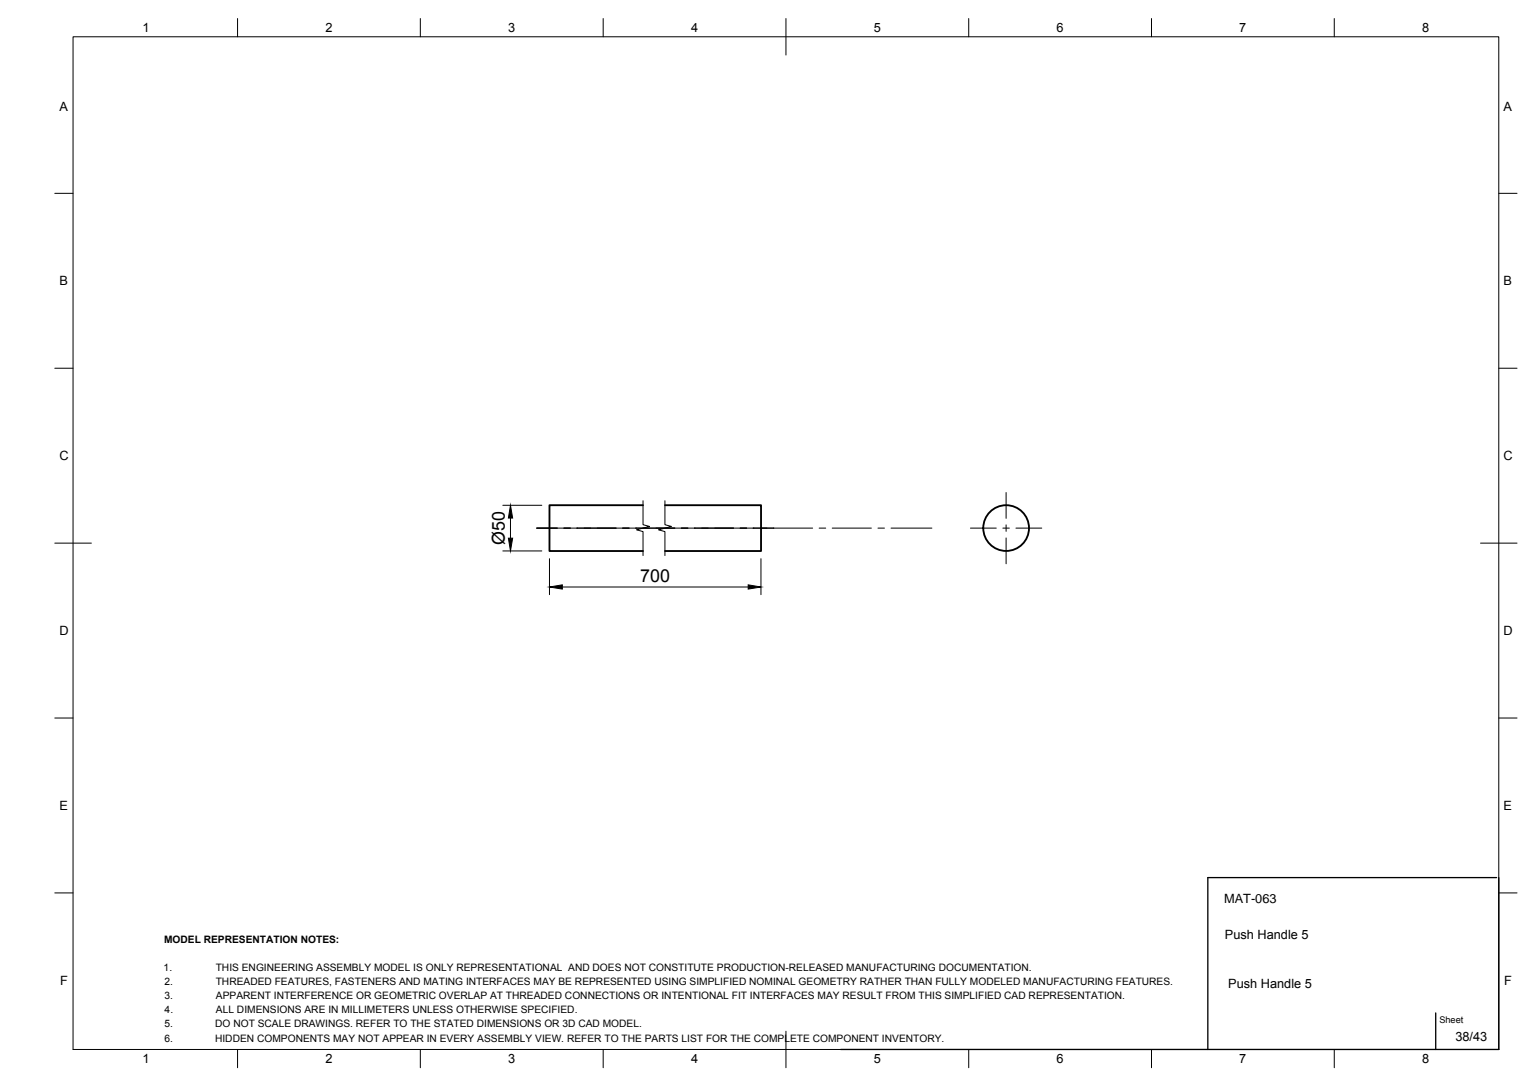
ISO-10303-21;
HEADER;
/* Generated by software containing ST-Developer
 * from STEP Tools, Inc. (www.steptools.com) 
 */

FILE_DESCRIPTION(
/* description */ (''),
/* implementation_level */ '2;1');

FILE_NAME(
/* name */ 'Push Handle 5.step',
/* time_stamp */ '2026-10-24T09:43:01-07:00',
/* author */ (''),
/* organization */ (''),
/* preprocessor_version */ 'ST-DEVELOPER v20.2',
/* originating_system */ 'Autodesk Translation Framework v15.15.0.0',
/* authorisation */ '');

FILE_SCHEMA (('AUTOMOTIVE_DESIGN { 1 0 10303 214 3 1 1 }'));
ENDSEC;

DATA;
#10=MECHANICAL_DESIGN_GEOMETRIC_PRESENTATION_REPRESENTATION('',(#301),#11112);
#235=SHAPE_REPRESENTATION_RELATIONSHIP('SRR','None',#11261,#268);
#268=ADVANCED_BREP_SHAPE_REPRESENTATION('',(#334),#11106);
#301=STYLED_ITEM('',(#11426),#334);
#334=MANIFOLD_SOLID_BREP('Push Handle 5',#6038);
#652=PLANE('',#7179);
#653=PLANE('',#7180);
#1010=FACE_OUTER_BOUND('',#1516,.T.);
#1011=FACE_OUTER_BOUND('',#1517,.T.);
#1012=FACE_OUTER_BOUND('',#1518,.T.);
#1516=EDGE_LOOP('',(#5403,#5404,#5405,#5406));
#1517=EDGE_LOOP('',(#5407));
#1518=EDGE_LOOP('',(#5408));
#1897=LINE('',#10903,#2256);
#2256=VECTOR('',#9141,0.025);
#2654=CIRCLE('',#7177,0.025);
#2655=CIRCLE('',#7178,0.025);
#3148=VERTEX_POINT('',#10900);
#3149=VERTEX_POINT('',#10902);
#3905=EDGE_CURVE('',#3148,#3148,#2654,.F.);
#3906=EDGE_CURVE('',#3148,#3149,#1897,.T.);
#3907=EDGE_CURVE('',#3149,#3149,#2655,.T.);
#5403=ORIENTED_EDGE('',*,*,#3905,.T.);
#5404=ORIENTED_EDGE('',*,*,#3906,.T.);
#5405=ORIENTED_EDGE('',*,*,#3907,.T.);
#5406=ORIENTED_EDGE('',*,*,#3906,.F.);
#5407=ORIENTED_EDGE('',*,*,#3907,.F.);
#5408=ORIENTED_EDGE('',*,*,#3905,.F.);
#5632=CYLINDRICAL_SURFACE('',#7176,0.025);
#5983=ADVANCED_FACE('',(#1010),#5632,.T.);
#5984=ADVANCED_FACE('',(#1011),#652,.T.);
#5985=ADVANCED_FACE('',(#1012),#653,.F.);
#6038=CLOSED_SHELL('',(#5983,#5984,#5985));
#7175=AXIS2_PLACEMENT_3D('',#10898,#9135,#9136);
#7176=AXIS2_PLACEMENT_3D('',#10899,#9137,#9138);
#7177=AXIS2_PLACEMENT_3D('',#10901,#9139,#9140);
#7178=AXIS2_PLACEMENT_3D('',#10904,#9142,#9143);
#7179=AXIS2_PLACEMENT_3D('',#10905,#9144,#9145);
#7180=AXIS2_PLACEMENT_3D('',#10906,#9146,#9147);
#9135=DIRECTION('axis',(0.,0.,1.));
#9136=DIRECTION('refdir',(1.,0.,0.));
#9137=DIRECTION('center_axis',(-1.,0.,0.));
#9138=DIRECTION('ref_axis',(0.,0.,1.));
#9139=DIRECTION('center_axis',(-1.,0.,0.));
#9140=DIRECTION('ref_axis',(0.,0.,1.));
#9141=DIRECTION('',(1.,0.,0.));
#9142=DIRECTION('center_axis',(-1.,0.,0.));
#9143=DIRECTION('ref_axis',(0.,0.,1.));
#9144=DIRECTION('center_axis',(1.,1.14194368292889E-16,-1.4591502616446E-16));
#9145=DIRECTION('ref_axis',(-1.4591502616446E-16,0.,-1.));
#9146=DIRECTION('center_axis',(1.,-1.14194368292889E-16,1.4591502616446E-16));
#9147=DIRECTION('ref_axis',(1.4591502616446E-16,0.,-1.));
#10898=CARTESIAN_POINT('',(0.,0.,0.));
#10899=CARTESIAN_POINT('Origin',(0.35,0.69,-1.3));
#10900=CARTESIAN_POINT('',(-0.35,0.69,-1.325));
#10901=CARTESIAN_POINT('Origin',(-0.35,0.69,-1.3));
#10902=CARTESIAN_POINT('',(0.35,0.69,-1.325));
#10903=CARTESIAN_POINT('',(0.35,0.69,-1.325));
#10904=CARTESIAN_POINT('Origin',(0.35,0.69,-1.3));
#10905=CARTESIAN_POINT('Origin',(0.35,0.69,-1.3));
#10906=CARTESIAN_POINT('Origin',(-0.35,0.69,-1.3));
#11067=UNCERTAINTY_MEASURE_WITH_UNIT(LENGTH_MEASURE(1.E-5),#11113,
'DISTANCE_ACCURACY_VALUE',
'Maximum model space distance between geometric entities at asserted c
onnectivities');
#11073=UNCERTAINTY_MEASURE_WITH_UNIT(LENGTH_MEASURE(1.E-5),#11113,
'DISTANCE_ACCURACY_VALUE',
'Maximum model space distance between geometric entities at asserted c
onnectivities');
#11106=(
GEOMETRIC_REPRESENTATION_CONTEXT(3)
GLOBAL_UNCERTAINTY_ASSIGNED_CONTEXT((#11067))
GLOBAL_UNIT_ASSIGNED_CONTEXT((#11113,#11114,#11115))
REPRESENTATION_CONTEXT('','3D')
);
#11112=(
GEOMETRIC_REPRESENTATION_CONTEXT(3)
GLOBAL_UNCERTAINTY_ASSIGNED_CONTEXT((#11073))
GLOBAL_UNIT_ASSIGNED_CONTEXT((#11113,#11114,#11115))
REPRESENTATION_CONTEXT('','3D')
);
#11113=(
LENGTH_UNIT()
NAMED_UNIT(*)
SI_UNIT($,.METRE.)
);
#11114=(
NAMED_UNIT(*)
PLANE_ANGLE_UNIT()
SI_UNIT($,.RADIAN.)
);
#11115=(
NAMED_UNIT(*)
SI_UNIT($,.STERADIAN.)
SOLID_ANGLE_UNIT()
);
#11148=SHAPE_DEFINITION_REPRESENTATION(#11199,#11261);
#11199=PRODUCT_DEFINITION_SHAPE('',$,#11300);
#11261=SHAPE_REPRESENTATION('',(#7175),#11106);
#11267=PRODUCT_DEFINITION_CONTEXT('part definition',#11383,'design');
#11300=PRODUCT_DEFINITION('Push Handle 5','Push Handle 5',#11338,#11267);
#11338=PRODUCT_DEFINITION_FORMATION('',$,#11417);
#11383=APPLICATION_CONTEXT(
'Core Data for Automotive Mechanical Design Process');
#11384=PRODUCT_CONTEXT('part definition',#11383,'mechanical');
#11417=PRODUCT('Push Handle 5','Push Handle 5',
'back_push__ DE     2477',(#11384));
#11426=PRESENTATION_STYLE_ASSIGNMENT((#11430));
#11430=SURFACE_STYLE_USAGE(.BOTH.,#11434);
#11434=SURFACE_SIDE_STYLE('',(#11438));
#11438=SURFACE_STYLE_FILL_AREA(#11442);
#11442=FILL_AREA_STYLE('Opaque(202,209,238)',(#11446));
#11446=FILL_AREA_STYLE_COLOUR('Opaque(202,209,238)',#11450);
#11450=COLOUR_RGB('Opaque(202,209,238)',0.792156862745098,0.819607843137255,
0.933333333333333);
ENDSEC;
END-ISO-10303-21;
